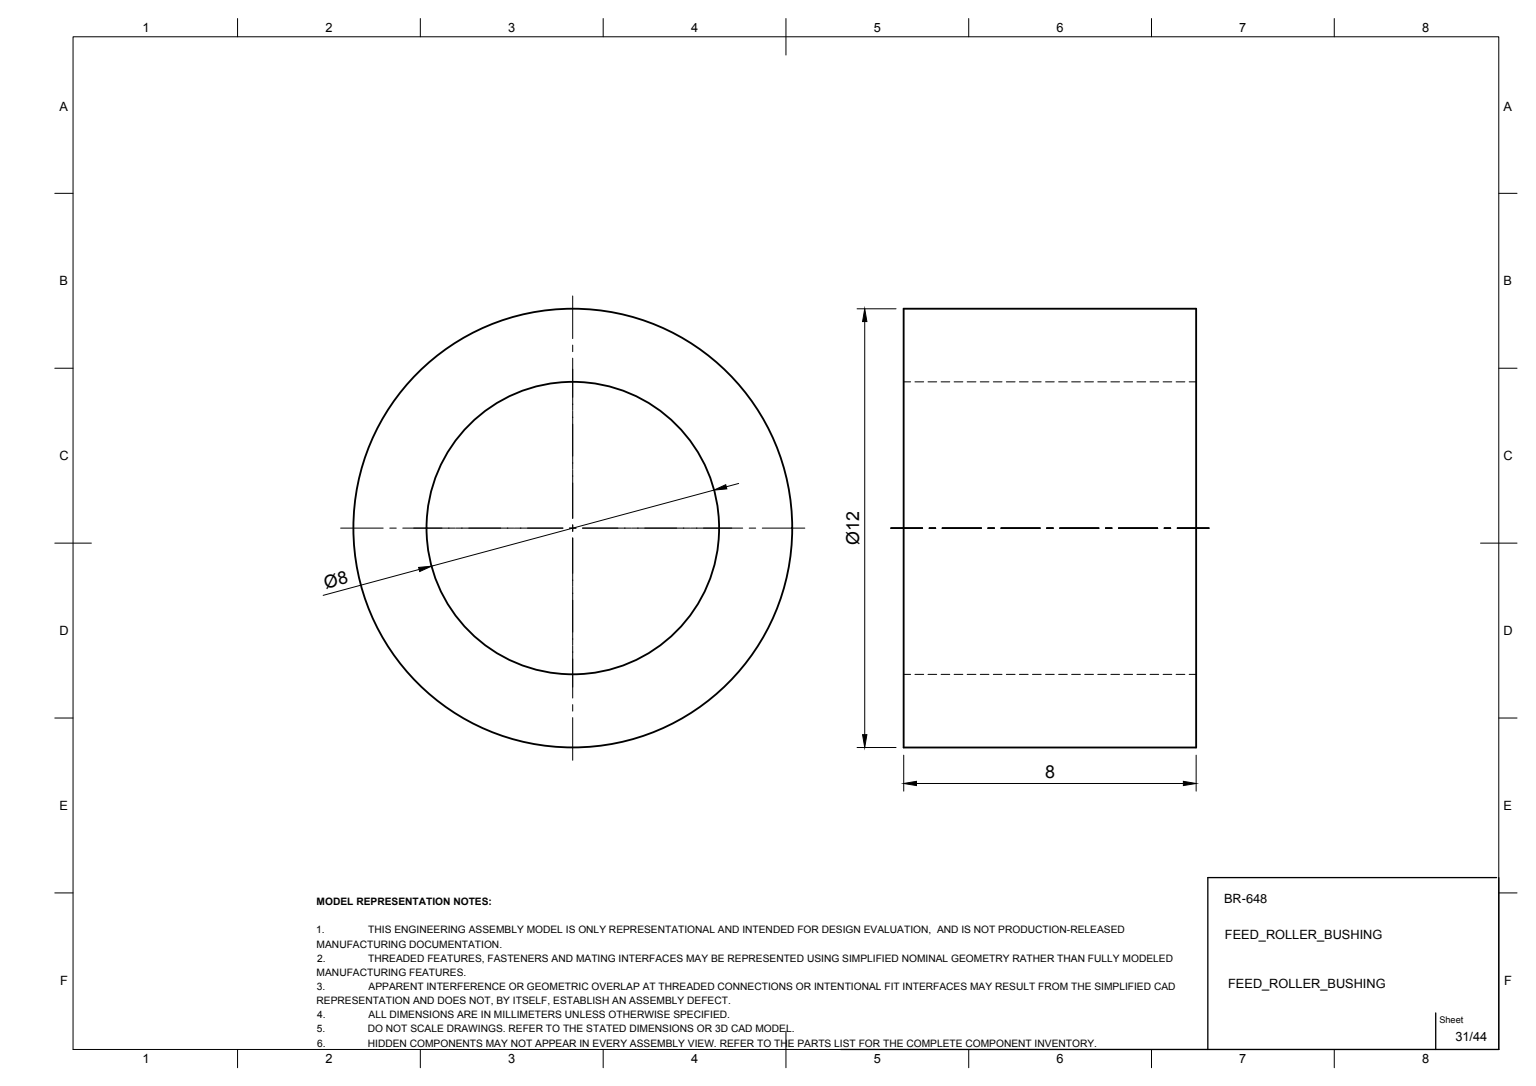
ISO-10303-21;
HEADER;
FILE_DESCRIPTION((''),'2;1');
FILE_NAME('FEED_ROLLER_BUSHING.step','2026-10-01T22:05:39-07:00',(''),(''),'','','');
FILE_SCHEMA (('AUTOMOTIVE_DESIGN { 1 0 10303 214 3 1 1 }'));
ENDSEC;
DATA;
#10=MECHANICAL_DESIGN_GEOMETRIC_PRESENTATION_REPRESENTATION('',(#629),#24628);
#545=SHAPE_REPRESENTATION_RELATIONSHIP('SRR','None',#24818,#587) ;
#587=ADVANCED_BREP_SHAPE_REPRESENTATION('',(#668),#24608) ;
#629=STYLED_ITEM('',(#25039),#668) ;
#668=MANIFOLD_SOLID_BREP('FEED_ROLLER_BUSHING',#13171) ;
#886=FACE_BOUND('',#4496,.T.) ;
#887=FACE_BOUND('',#4498,.T.) ;
#1560=LINE('',#23295,#2396) ;
#1561=LINE('',#23301,#2397) ;
#2396=VECTOR('',#18649,0.4) ;
#2397=VECTOR('',#18656,0.6) ;
#2898=CYLINDRICAL_SURFACE('',#15000,0.4) ;
#2899=CYLINDRICAL_SURFACE('',#15003,0.6) ;
#3526=FACE_OUTER_BOUND('',#4493,.T.) ;
#3527=FACE_OUTER_BOUND('',#4494,.T.) ;
#3528=FACE_OUTER_BOUND('',#4495,.T.) ;
#3529=FACE_OUTER_BOUND('',#4497,.T.) ;
#4493=EDGE_LOOP('',(#11135,#11136,#11137,#11138)) ;
#4494=EDGE_LOOP('',(#11139,#11140,#11141,#11142)) ;
#4495=EDGE_LOOP('',(#11143)) ;
#4496=EDGE_LOOP('',(#11144)) ;
#4497=EDGE_LOOP('',(#11145)) ;
#4498=EDGE_LOOP('',(#11146)) ;
#5407=CIRCLE('',#15001,0.4) ;
#5408=CIRCLE('',#15002,0.4) ;
#5409=CIRCLE('',#15004,0.6) ;
#5410=CIRCLE('',#15005,0.6) ;
#6449=VERTEX_POINT('',#23292) ;
#6450=VERTEX_POINT('',#23294) ;
#6451=VERTEX_POINT('',#23298) ;
#6452=VERTEX_POINT('',#23300) ;
#8057=EDGE_CURVE('',#6449,#6449,#5407,.T.) ;
#8058=EDGE_CURVE('',#6449,#6450,#1560,.T.) ;
#8059=EDGE_CURVE('',#6450,#6450,#5408,.T.) ;
#8060=EDGE_CURVE('',#6451,#6451,#5409,.T.) ;
#8061=EDGE_CURVE('',#6451,#6452,#1561,.T.) ;
#8062=EDGE_CURVE('',#6452,#6452,#5410,.T.) ;
#11135=ORIENTED_EDGE('',*,*,#8057,.F.) ;
#11136=ORIENTED_EDGE('',*,*,#8058,.T.) ;
#11137=ORIENTED_EDGE('',*,*,#8059,.F.) ;
#11138=ORIENTED_EDGE('',*,*,#8058,.F.) ;
#11139=ORIENTED_EDGE('',*,*,#8060,.F.) ;
#11140=ORIENTED_EDGE('',*,*,#8061,.T.) ;
#11141=ORIENTED_EDGE('',*,*,#8062,.F.) ;
#11142=ORIENTED_EDGE('',*,*,#8061,.F.) ;
#11143=ORIENTED_EDGE('',*,*,#8062,.T.) ;
#11144=ORIENTED_EDGE('',*,*,#8057,.T.) ;
#11145=ORIENTED_EDGE('',*,*,#8060,.T.) ;
#11146=ORIENTED_EDGE('',*,*,#8059,.T.) ;
#12213=PLANE('',#15006) ;
#12214=PLANE('',#15007) ;
#12921=ADVANCED_FACE('',(#3526),#2898,.F.) ;
#12922=ADVANCED_FACE('',(#3527),#2899,.T.) ;
#12923=ADVANCED_FACE('',(#3528,#886),#12213,.T.) ;
#12924=ADVANCED_FACE('',(#3529,#887),#12214,.T.) ;
#13171=CLOSED_SHELL('',(#12921,#12922,#12923,#12924)) ;
#14999=AXIS2_PLACEMENT_3D('',#23290,#18643,#18644) ;
#15000=AXIS2_PLACEMENT_3D('',#23291,#18645,#18646) ;
#15001=AXIS2_PLACEMENT_3D('',#23293,#18647,#18648) ;
#15002=AXIS2_PLACEMENT_3D('',#23296,#18650,#18651) ;
#15003=AXIS2_PLACEMENT_3D('',#23297,#18652,#18653) ;
#15004=AXIS2_PLACEMENT_3D('',#23299,#18654,#18655) ;
#15005=AXIS2_PLACEMENT_3D('',#23302,#18657,#18658) ;
#15006=AXIS2_PLACEMENT_3D('',#23303,#18659,#18660) ;
#15007=AXIS2_PLACEMENT_3D('',#23304,#18661,#18662) ;
#18643=DIRECTION('axis',(0.,0.,1.)) ;
#18644=DIRECTION('refdir',(1.,0.,0.)) ;
#18645=DIRECTION('center_axis',(0.,1.,0.)) ;
#18646=DIRECTION('ref_axis',(1.,0.,0.)) ;
#18647=DIRECTION('center_axis',(0.,1.,0.)) ;
#18648=DIRECTION('ref_axis',(1.,0.,0.)) ;
#18649=DIRECTION('',(0.,1.,0.)) ;
#18650=DIRECTION('center_axis',(0.,-1.,0.)) ;
#18651=DIRECTION('ref_axis',(1.,0.,0.)) ;
#18652=DIRECTION('center_axis',(0.,1.,0.)) ;
#18653=DIRECTION('ref_axis',(1.,0.,0.)) ;
#18654=DIRECTION('center_axis',(0.,1.,0.)) ;
#18655=DIRECTION('ref_axis',(1.,0.,0.)) ;
#18656=DIRECTION('',(0.,-1.,0.)) ;
#18657=DIRECTION('center_axis',(0.,-1.,0.)) ;
#18658=DIRECTION('ref_axis',(1.,0.,0.)) ;
#18659=DIRECTION('center_axis',(0.,-1.,0.)) ;
#18660=DIRECTION('ref_axis',(-1.,0.,0.)) ;
#18661=DIRECTION('center_axis',(0.,1.,0.)) ;
#18662=DIRECTION('ref_axis',(1.,0.,0.)) ;
#23290=CARTESIAN_POINT('',(0.,0.,0.)) ;
#23291=CARTESIAN_POINT('Origin',(-23.,-4.4,-2.2)) ;
#23292=CARTESIAN_POINT('',(-23.4,-4.8,-2.2)) ;
#23293=CARTESIAN_POINT('Origin',(-23.,-4.8,-2.2)) ;
#23294=CARTESIAN_POINT('',(-23.4,-4.,-2.2)) ;
#23295=CARTESIAN_POINT('',(-23.4,-4.4,-2.2)) ;
#23296=CARTESIAN_POINT('Origin',(-23.,-4.,-2.2)) ;
#23297=CARTESIAN_POINT('Origin',(-23.,-4.4,-2.2)) ;
#23298=CARTESIAN_POINT('',(-23.6,-4.,-2.2)) ;
#23299=CARTESIAN_POINT('Origin',(-23.,-4.,-2.2)) ;
#23300=CARTESIAN_POINT('',(-23.6,-4.8,-2.2)) ;
#23301=CARTESIAN_POINT('',(-23.6,-4.4,-2.2)) ;
#23302=CARTESIAN_POINT('Origin',(-23.,-4.8,-2.2)) ;
#23303=CARTESIAN_POINT('Origin',(-23.,-4.8,-2.2)) ;
#23304=CARTESIAN_POINT('Origin',(-23.,-4.,-2.2)) ;
#24560=UNCERTAINTY_MEASURE_WITH_UNIT(LENGTH_MEASURE(0.001),#24629,
'DISTANCE_ACCURACY_VALUE',
'Maximum model space distance between geometric entities at asserted c
onnectivities') ;
#24580=UNCERTAINTY_MEASURE_WITH_UNIT(LENGTH_MEASURE(0.001),#24629,
'DISTANCE_ACCURACY_VALUE',
'Maximum model space distance between geometric entities at asserted c
onnectivities') ;
#24608=(
GEOMETRIC_REPRESENTATION_CONTEXT(3)
GLOBAL_UNCERTAINTY_ASSIGNED_CONTEXT((#24560))
GLOBAL_UNIT_ASSIGNED_CONTEXT((#24629,#24631,#24632))
REPRESENTATION_CONTEXT('','3D')
) ;
#24628=(
GEOMETRIC_REPRESENTATION_CONTEXT(3)
GLOBAL_UNCERTAINTY_ASSIGNED_CONTEXT((#24580))
GLOBAL_UNIT_ASSIGNED_CONTEXT((#24629,#24631,#24632))
REPRESENTATION_CONTEXT('','3D')
) ;
#24629=(
LENGTH_UNIT()
NAMED_UNIT(*)
SI_UNIT(.CENTI.,.METRE.)
) ;
#24631=(
NAMED_UNIT(*)
PLANE_ANGLE_UNIT()
SI_UNIT($,.RADIAN.)
) ;
#24632=(
NAMED_UNIT(*)
SI_UNIT($,.STERADIAN.)
SOLID_ANGLE_UNIT()
) ;
#24660=SHAPE_DEFINITION_REPRESENTATION(#24729,#24818) ;
#24729=PRODUCT_DEFINITION_SHAPE('',$,#24866) ;
#24818=SHAPE_REPRESENTATION('',(#14999),#24608) ;
#24838=PRODUCT_DEFINITION_CONTEXT('part definition',#24981,'design') ;
#24866=PRODUCT_DEFINITION('FEED_ROLLER_BUSHING',
'FEED_ROLLER_BUSHING',#24913,#24838) ;
#24913=PRODUCT_DEFINITION_FORMATION('',$,#25010) ;
#24981=APPLICATION_CONTEXT(
'Core Data for Automotive Mechanical Design Process') ;
#24982=PRODUCT_CONTEXT('part definition',#24981,'mechanical') ;
#25010=PRODUCT('FEED_ROLLER_BUSHING','FEED_ROLLER_BUSHING',$,(#24982)) ;
#25039=PRESENTATION_STYLE_ASSIGNMENT((#25049)) ;
#25049=SURFACE_STYLE_USAGE(.BOTH.,#25059) ;
#25059=SURFACE_SIDE_STYLE('',(#25069)) ;
#25069=SURFACE_STYLE_FILL_AREA(#25079) ;
#25079=FILL_AREA_STYLE('Brass - Polished',(#25089)) ;
#25089=FILL_AREA_STYLE_COLOUR('Brass - Polished',#25099) ;
#25099=COLOUR_RGB('Brass - Polished', 0.09019608, 0.27058824, 0.51372549) ;
ENDSEC;
END-ISO-10303-21;
